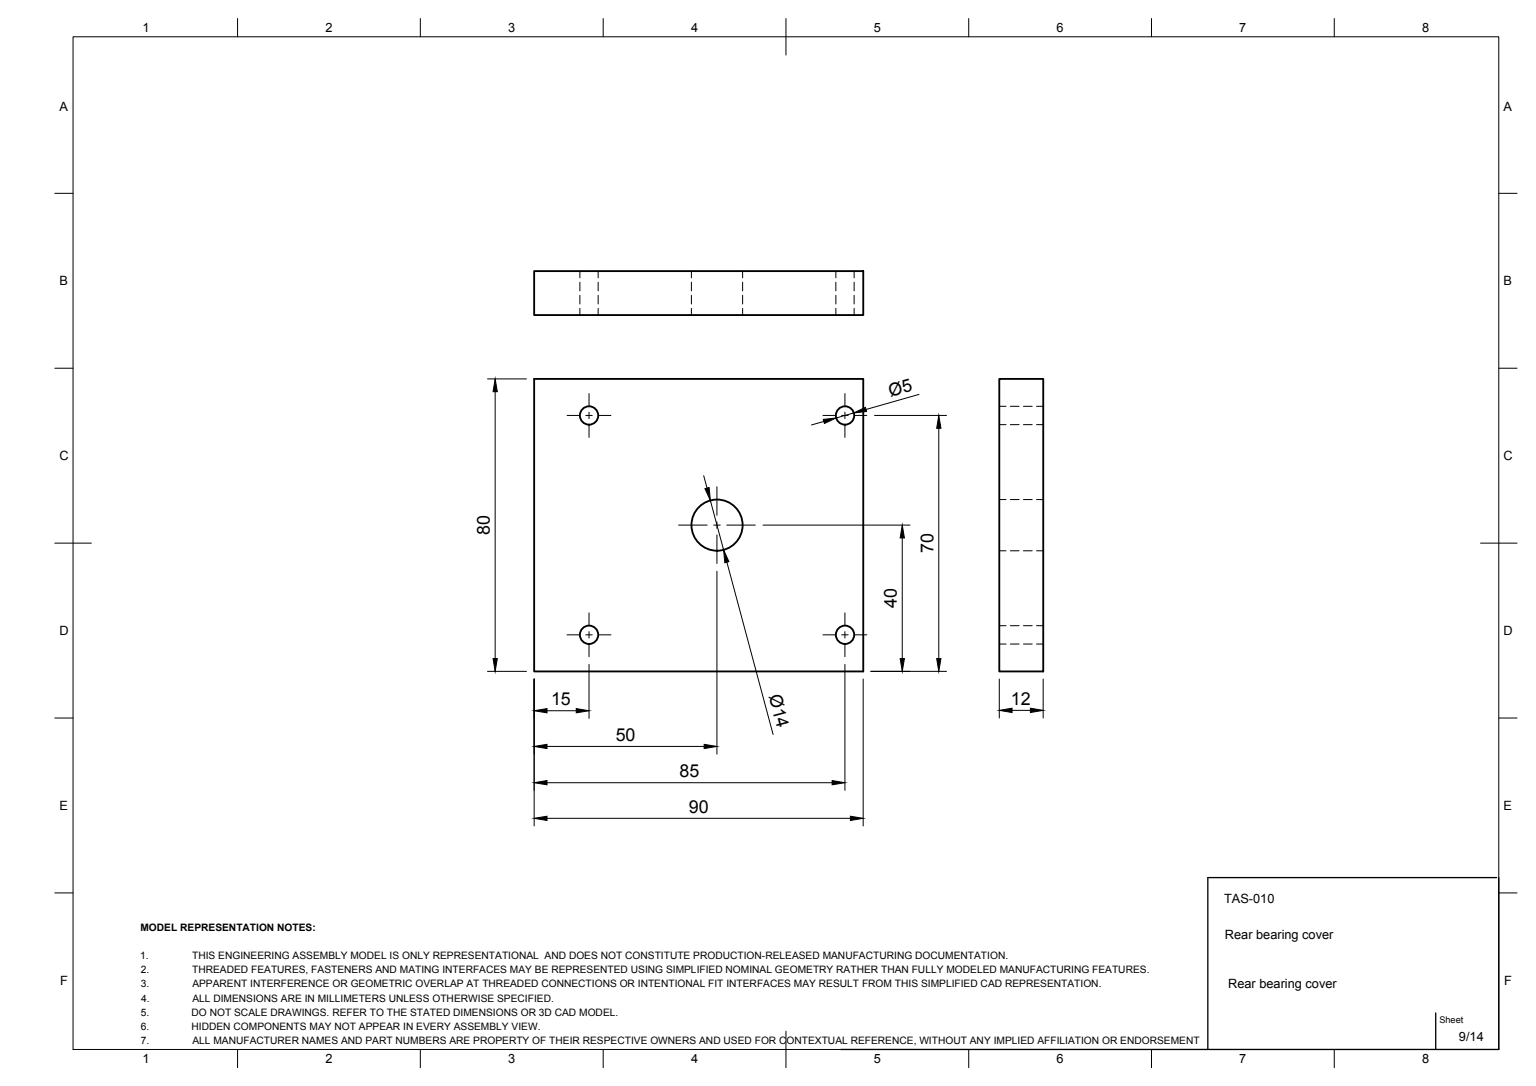
ISO-10303-21;
HEADER;
/* Generated by software containing ST-Developer
 * from STEP Tools, Inc. (www.steptools.com) 
 */

FILE_DESCRIPTION(
/* description */ (
'Independent keyed-quill tailstock, native coupled50mm slider andM16x2
 feed screw, conical dead center, bronze sleeves/thrust washers, cross
-pinned handwheel and bolted guide key. Custom center taper; no standa
rd taper compatibility, machine-bed compatibility or load rating assig
ned.'),
/* implementation_level */ '2;1');

FILE_NAME(
/* name */ 'Rear bearing cover.step',
/* time_stamp */ '2026-11-14T07:17:36-08:00',
/* author */ (''),
/* organization */ (''),
/* preprocessor_version */ 'ST-DEVELOPER v20.2',
/* originating_system */ 'Autodesk Translation Framework v15.17.0.0',
/* authorisation */ '');

FILE_SCHEMA (('AUTOMOTIVE_DESIGN { 1 0 10303 214 3 1 1 }'));
ENDSEC;

DATA;
#10=MECHANICAL_DESIGN_GEOMETRIC_PRESENTATION_REPRESENTATION('',(#159),#289387);
#125=SHAPE_REPRESENTATION_RELATIONSHIP('SRR','None',#289460,#142);
#142=ADVANCED_BREP_SHAPE_REPRESENTATION('',(#176),#289376);
#159=STYLED_ITEM('',(#289552),#176);
#176=MANIFOLD_SOLID_BREP('Body1',#16847);
#228=FACE_BOUND('',#1545,.T.);
#229=FACE_BOUND('',#1546,.T.);
#230=FACE_BOUND('',#1547,.T.);
#231=FACE_BOUND('',#1548,.T.);
#232=FACE_BOUND('',#1549,.T.);
#233=FACE_BOUND('',#1558,.T.);
#234=FACE_BOUND('',#1559,.T.);
#235=FACE_BOUND('',#1560,.T.);
#236=FACE_BOUND('',#1561,.T.);
#237=FACE_BOUND('',#1562,.T.);
#365=PLANE('',#17554);
#366=PLANE('',#17555);
#367=PLANE('',#17556);
#368=PLANE('',#17572);
#369=PLANE('',#17573);
#370=PLANE('',#17574);
#851=FACE_OUTER_BOUND('',#1542,.T.);
#852=FACE_OUTER_BOUND('',#1543,.T.);
#853=FACE_OUTER_BOUND('',#1544,.T.);
#854=FACE_OUTER_BOUND('',#1550,.T.);
#855=FACE_OUTER_BOUND('',#1551,.T.);
#856=FACE_OUTER_BOUND('',#1552,.T.);
#857=FACE_OUTER_BOUND('',#1553,.T.);
#858=FACE_OUTER_BOUND('',#1554,.T.);
#859=FACE_OUTER_BOUND('',#1555,.T.);
#860=FACE_OUTER_BOUND('',#1556,.T.);
#861=FACE_OUTER_BOUND('',#1557,.T.);
#1542=EDGE_LOOP('',(#13733,#13734,#13735,#13736));
#1543=EDGE_LOOP('',(#13737,#13738,#13739,#13740));
#1544=EDGE_LOOP('',(#13741,#13742,#13743,#13744));
#1545=EDGE_LOOP('',(#13745));
#1546=EDGE_LOOP('',(#13746));
#1547=EDGE_LOOP('',(#13747));
#1548=EDGE_LOOP('',(#13748));
#1549=EDGE_LOOP('',(#13749));
#1550=EDGE_LOOP('',(#13750,#13751,#13752,#13753));
#1551=EDGE_LOOP('',(#13754,#13755,#13756,#13757));
#1552=EDGE_LOOP('',(#13758,#13759,#13760,#13761));
#1553=EDGE_LOOP('',(#13762,#13763,#13764,#13765));
#1554=EDGE_LOOP('',(#13766,#13767,#13768,#13769));
#1555=EDGE_LOOP('',(#13770,#13771,#13772,#13773));
#1556=EDGE_LOOP('',(#13774,#13775,#13776,#13777));
#1557=EDGE_LOOP('',(#13778,#13779,#13780,#13781));
#1558=EDGE_LOOP('',(#13782));
#1559=EDGE_LOOP('',(#13783));
#1560=EDGE_LOOP('',(#13784));
#1561=EDGE_LOOP('',(#13785));
#1562=EDGE_LOOP('',(#13786));
#1903=CIRCLE('',#17557,2.5);
#1904=CIRCLE('',#17558,2.5);
#1905=CIRCLE('',#17559,2.5);
#1906=CIRCLE('',#17560,2.5);
#1907=CIRCLE('',#17561,7.);
#1908=CIRCLE('',#17563,2.5);
#1909=CIRCLE('',#17565,2.5);
#1910=CIRCLE('',#17567,2.5);
#1911=CIRCLE('',#17569,2.5);
#1912=CIRCLE('',#17571,7.);
#4355=LINE('',#185232,#4992);
#4356=LINE('',#185234,#4993);
#4357=LINE('',#185236,#4994);
#4358=LINE('',#185237,#4995);
#4359=LINE('',#185240,#4996);
#4360=LINE('',#185242,#4997);
#4361=LINE('',#185243,#4998);
#4362=LINE('',#185246,#4999);
#4363=LINE('',#185247,#5000);
#4364=LINE('',#185261,#5001);
#4365=LINE('',#185265,#5002);
#4366=LINE('',#185269,#5003);
#4367=LINE('',#185273,#5004);
#4368=LINE('',#185277,#5005);
#4369=LINE('',#185280,#5006);
#4370=LINE('',#185281,#5007);
#4371=LINE('',#185283,#5008);
#4992=VECTOR('',#19321,10.);
#4993=VECTOR('',#19322,10.);
#4994=VECTOR('',#19323,10.);
#4995=VECTOR('',#19324,10.);
#4996=VECTOR('',#19327,10.);
#4997=VECTOR('',#19328,10.);
#4998=VECTOR('',#19329,10.);
#4999=VECTOR('',#19332,10.);
#5000=VECTOR('',#19333,10.);
#5001=VECTOR('',#19348,2.5);
#5002=VECTOR('',#19353,2.5);
#5003=VECTOR('',#19358,2.5);
#5004=VECTOR('',#19363,2.5);
#5005=VECTOR('',#19368,7.);
#5006=VECTOR('',#19371,10.);
#5007=VECTOR('',#19372,10.);
#5008=VECTOR('',#19375,10.);
#6600=VERTEX_POINT('',#185230);
#6601=VERTEX_POINT('',#185231);
#6602=VERTEX_POINT('',#185233);
#6603=VERTEX_POINT('',#185235);
#6604=VERTEX_POINT('',#185239);
#6605=VERTEX_POINT('',#185241);
#6606=VERTEX_POINT('',#185245);
#6607=VERTEX_POINT('',#185248);
#6608=VERTEX_POINT('',#185250);
#6609=VERTEX_POINT('',#185252);
#6610=VERTEX_POINT('',#185254);
#6611=VERTEX_POINT('',#185256);
#6612=VERTEX_POINT('',#185259);
#6613=VERTEX_POINT('',#185263);
#6614=VERTEX_POINT('',#185267);
#6615=VERTEX_POINT('',#185271);
#6616=VERTEX_POINT('',#185275);
#6617=VERTEX_POINT('',#185279);
#9178=EDGE_CURVE('',#6600,#6601,#4355,.T.);
#9179=EDGE_CURVE('',#6602,#6600,#4356,.T.);
#9180=EDGE_CURVE('',#6603,#6602,#4357,.T.);
#9181=EDGE_CURVE('',#6601,#6603,#4358,.T.);
#9182=EDGE_CURVE('',#6603,#6604,#4359,.T.);
#9183=EDGE_CURVE('',#6604,#6605,#4360,.T.);
#9184=EDGE_CURVE('',#6601,#6605,#4361,.T.);
#9185=EDGE_CURVE('',#6606,#6602,#4362,.T.);
#9186=EDGE_CURVE('',#6604,#6606,#4363,.T.);
#9187=EDGE_CURVE('',#6607,#6607,#1903,.T.);
#9188=EDGE_CURVE('',#6608,#6608,#1904,.T.);
#9189=EDGE_CURVE('',#6609,#6609,#1905,.T.);
#9190=EDGE_CURVE('',#6610,#6610,#1906,.T.);
#9191=EDGE_CURVE('',#6611,#6611,#1907,.T.);
#9192=EDGE_CURVE('',#6612,#6612,#1908,.T.);
#9193=EDGE_CURVE('',#6612,#6607,#4364,.T.);
#9194=EDGE_CURVE('',#6613,#6613,#1909,.T.);
#9195=EDGE_CURVE('',#6613,#6608,#4365,.T.);
#9196=EDGE_CURVE('',#6614,#6614,#1910,.T.);
#9197=EDGE_CURVE('',#6614,#6609,#4366,.T.);
#9198=EDGE_CURVE('',#6615,#6615,#1911,.T.);
#9199=EDGE_CURVE('',#6615,#6610,#4367,.T.);
#9200=EDGE_CURVE('',#6616,#6616,#1912,.T.);
#9201=EDGE_CURVE('',#6616,#6611,#4368,.T.);
#9202=EDGE_CURVE('',#6606,#6617,#4369,.T.);
#9203=EDGE_CURVE('',#6605,#6617,#4370,.T.);
#9204=EDGE_CURVE('',#6617,#6600,#4371,.T.);
#13733=ORIENTED_EDGE('',*,*,#9178,.F.);
#13734=ORIENTED_EDGE('',*,*,#9179,.F.);
#13735=ORIENTED_EDGE('',*,*,#9180,.F.);
#13736=ORIENTED_EDGE('',*,*,#9181,.F.);
#13737=ORIENTED_EDGE('',*,*,#9181,.T.);
#13738=ORIENTED_EDGE('',*,*,#9182,.T.);
#13739=ORIENTED_EDGE('',*,*,#9183,.T.);
#13740=ORIENTED_EDGE('',*,*,#9184,.F.);
#13741=ORIENTED_EDGE('',*,*,#9180,.T.);
#13742=ORIENTED_EDGE('',*,*,#9185,.F.);
#13743=ORIENTED_EDGE('',*,*,#9186,.F.);
#13744=ORIENTED_EDGE('',*,*,#9182,.F.);
#13745=ORIENTED_EDGE('',*,*,#9187,.T.);
#13746=ORIENTED_EDGE('',*,*,#9188,.T.);
#13747=ORIENTED_EDGE('',*,*,#9189,.T.);
#13748=ORIENTED_EDGE('',*,*,#9190,.T.);
#13749=ORIENTED_EDGE('',*,*,#9191,.T.);
#13750=ORIENTED_EDGE('',*,*,#9192,.F.);
#13751=ORIENTED_EDGE('',*,*,#9193,.T.);
#13752=ORIENTED_EDGE('',*,*,#9187,.F.);
#13753=ORIENTED_EDGE('',*,*,#9193,.F.);
#13754=ORIENTED_EDGE('',*,*,#9194,.F.);
#13755=ORIENTED_EDGE('',*,*,#9195,.T.);
#13756=ORIENTED_EDGE('',*,*,#9188,.F.);
#13757=ORIENTED_EDGE('',*,*,#9195,.F.);
#13758=ORIENTED_EDGE('',*,*,#9196,.F.);
#13759=ORIENTED_EDGE('',*,*,#9197,.T.);
#13760=ORIENTED_EDGE('',*,*,#9189,.F.);
#13761=ORIENTED_EDGE('',*,*,#9197,.F.);
#13762=ORIENTED_EDGE('',*,*,#9198,.F.);
#13763=ORIENTED_EDGE('',*,*,#9199,.T.);
#13764=ORIENTED_EDGE('',*,*,#9190,.F.);
#13765=ORIENTED_EDGE('',*,*,#9199,.F.);
#13766=ORIENTED_EDGE('',*,*,#9200,.F.);
#13767=ORIENTED_EDGE('',*,*,#9201,.T.);
#13768=ORIENTED_EDGE('',*,*,#9191,.F.);
#13769=ORIENTED_EDGE('',*,*,#9201,.F.);
#13770=ORIENTED_EDGE('',*,*,#9186,.T.);
#13771=ORIENTED_EDGE('',*,*,#9202,.T.);
#13772=ORIENTED_EDGE('',*,*,#9203,.F.);
#13773=ORIENTED_EDGE('',*,*,#9183,.F.);
#13774=ORIENTED_EDGE('',*,*,#9179,.T.);
#13775=ORIENTED_EDGE('',*,*,#9204,.F.);
#13776=ORIENTED_EDGE('',*,*,#9202,.F.);
#13777=ORIENTED_EDGE('',*,*,#9185,.T.);
#13778=ORIENTED_EDGE('',*,*,#9178,.T.);
#13779=ORIENTED_EDGE('',*,*,#9184,.T.);
#13780=ORIENTED_EDGE('',*,*,#9203,.T.);
#13781=ORIENTED_EDGE('',*,*,#9204,.T.);
#13782=ORIENTED_EDGE('',*,*,#9200,.T.);
#13783=ORIENTED_EDGE('',*,*,#9198,.T.);
#13784=ORIENTED_EDGE('',*,*,#9196,.T.);
#13785=ORIENTED_EDGE('',*,*,#9194,.T.);
#13786=ORIENTED_EDGE('',*,*,#9192,.T.);
#16040=CYLINDRICAL_SURFACE('',#17562,2.5);
#16041=CYLINDRICAL_SURFACE('',#17564,2.5);
#16042=CYLINDRICAL_SURFACE('',#17566,2.5);
#16043=CYLINDRICAL_SURFACE('',#17568,2.5);
#16044=CYLINDRICAL_SURFACE('',#17570,7.);
#16619=ADVANCED_FACE('',(#851),#365,.F.);
#16620=ADVANCED_FACE('',(#852),#366,.T.);
#16621=ADVANCED_FACE('',(#853,#228,#229,#230,#231,#232),#367,.F.);
#16622=ADVANCED_FACE('',(#854),#16040,.F.);
#16623=ADVANCED_FACE('',(#855),#16041,.F.);
#16624=ADVANCED_FACE('',(#856),#16042,.F.);
#16625=ADVANCED_FACE('',(#857),#16043,.F.);
#16626=ADVANCED_FACE('',(#858),#16044,.F.);
#16627=ADVANCED_FACE('',(#859),#368,.T.);
#16628=ADVANCED_FACE('',(#860),#369,.T.);
#16629=ADVANCED_FACE('',(#861,#233,#234,#235,#236,#237),#370,.T.);
#16847=CLOSED_SHELL('',(#16619,#16620,#16621,#16622,#16623,#16624,#16625,
#16626,#16627,#16628,#16629));
#17553=AXIS2_PLACEMENT_3D('',#185228,#19317,#19318);
#17554=AXIS2_PLACEMENT_3D('',#185229,#19319,#19320);
#17555=AXIS2_PLACEMENT_3D('',#185238,#19325,#19326);
#17556=AXIS2_PLACEMENT_3D('',#185244,#19330,#19331);
#17557=AXIS2_PLACEMENT_3D('',#185249,#19334,#19335);
#17558=AXIS2_PLACEMENT_3D('',#185251,#19336,#19337);
#17559=AXIS2_PLACEMENT_3D('',#185253,#19338,#19339);
#17560=AXIS2_PLACEMENT_3D('',#185255,#19340,#19341);
#17561=AXIS2_PLACEMENT_3D('',#185257,#19342,#19343);
#17562=AXIS2_PLACEMENT_3D('',#185258,#19344,#19345);
#17563=AXIS2_PLACEMENT_3D('',#185260,#19346,#19347);
#17564=AXIS2_PLACEMENT_3D('',#185262,#19349,#19350);
#17565=AXIS2_PLACEMENT_3D('',#185264,#19351,#19352);
#17566=AXIS2_PLACEMENT_3D('',#185266,#19354,#19355);
#17567=AXIS2_PLACEMENT_3D('',#185268,#19356,#19357);
#17568=AXIS2_PLACEMENT_3D('',#185270,#19359,#19360);
#17569=AXIS2_PLACEMENT_3D('',#185272,#19361,#19362);
#17570=AXIS2_PLACEMENT_3D('',#185274,#19364,#19365);
#17571=AXIS2_PLACEMENT_3D('',#185276,#19366,#19367);
#17572=AXIS2_PLACEMENT_3D('',#185278,#19369,#19370);
#17573=AXIS2_PLACEMENT_3D('',#185282,#19373,#19374);
#17574=AXIS2_PLACEMENT_3D('',#185284,#19376,#19377);
#19317=DIRECTION('axis',(0.,0.,1.));
#19318=DIRECTION('refdir',(1.,0.,0.));
#19319=DIRECTION('center_axis',(0.,1.,0.));
#19320=DIRECTION('ref_axis',(1.,0.,0.));
#19321=DIRECTION('',(1.,0.,0.));
#19322=DIRECTION('',(0.,0.,1.));
#19323=DIRECTION('',(-1.,0.,0.));
#19324=DIRECTION('',(0.,0.,-1.));
#19325=DIRECTION('center_axis',(1.,0.,0.));
#19326=DIRECTION('ref_axis',(0.,1.,0.));
#19327=DIRECTION('',(0.,1.,0.));
#19328=DIRECTION('',(0.,0.,1.));
#19329=DIRECTION('',(0.,1.,0.));
#19330=DIRECTION('center_axis',(0.,0.,1.));
#19331=DIRECTION('ref_axis',(1.,0.,0.));
#19332=DIRECTION('',(0.,-1.,0.));
#19333=DIRECTION('',(-1.,0.,0.));
#19334=DIRECTION('center_axis',(0.,0.,1.));
#19335=DIRECTION('ref_axis',(1.,0.,0.));
#19336=DIRECTION('center_axis',(0.,0.,1.));
#19337=DIRECTION('ref_axis',(1.,0.,0.));
#19338=DIRECTION('center_axis',(0.,0.,1.));
#19339=DIRECTION('ref_axis',(1.,0.,0.));
#19340=DIRECTION('center_axis',(0.,0.,1.));
#19341=DIRECTION('ref_axis',(1.,0.,0.));
#19342=DIRECTION('center_axis',(0.,0.,1.));
#19343=DIRECTION('ref_axis',(1.,0.,0.));
#19344=DIRECTION('center_axis',(0.,0.,-1.));
#19345=DIRECTION('ref_axis',(1.,0.,0.));
#19346=DIRECTION('center_axis',(0.,0.,-1.));
#19347=DIRECTION('ref_axis',(1.,0.,0.));
#19348=DIRECTION('',(0.,0.,-1.));
#19349=DIRECTION('center_axis',(0.,0.,-1.));
#19350=DIRECTION('ref_axis',(1.,0.,0.));
#19351=DIRECTION('center_axis',(0.,0.,-1.));
#19352=DIRECTION('ref_axis',(1.,0.,0.));
#19353=DIRECTION('',(0.,0.,-1.));
#19354=DIRECTION('center_axis',(0.,0.,-1.));
#19355=DIRECTION('ref_axis',(1.,0.,0.));
#19356=DIRECTION('center_axis',(0.,0.,-1.));
#19357=DIRECTION('ref_axis',(1.,0.,0.));
#19358=DIRECTION('',(0.,0.,-1.));
#19359=DIRECTION('center_axis',(0.,0.,-1.));
#19360=DIRECTION('ref_axis',(1.,0.,0.));
#19361=DIRECTION('center_axis',(0.,0.,-1.));
#19362=DIRECTION('ref_axis',(1.,0.,0.));
#19363=DIRECTION('',(0.,0.,-1.));
#19364=DIRECTION('center_axis',(0.,0.,-1.));
#19365=DIRECTION('ref_axis',(1.,0.,0.));
#19366=DIRECTION('center_axis',(0.,0.,-1.));
#19367=DIRECTION('ref_axis',(1.,0.,0.));
#19368=DIRECTION('',(0.,0.,-1.));
#19369=DIRECTION('center_axis',(0.,1.,0.));
#19370=DIRECTION('ref_axis',(-1.,0.,0.));
#19371=DIRECTION('',(0.,0.,1.));
#19372=DIRECTION('',(-1.,0.,0.));
#19373=DIRECTION('center_axis',(-1.,0.,0.));
#19374=DIRECTION('ref_axis',(0.,-1.,0.));
#19375=DIRECTION('',(0.,-1.,0.));
#19376=DIRECTION('center_axis',(0.,0.,1.));
#19377=DIRECTION('ref_axis',(1.,0.,0.));
#185228=CARTESIAN_POINT('',(0.,0.,0.));
#185229=CARTESIAN_POINT('Origin',(-40.,-40.,12.));
#185230=CARTESIAN_POINT('',(-40.,-40.,12.));
#185231=CARTESIAN_POINT('',(40.,-40.,12.));
#185232=CARTESIAN_POINT('',(-20.,-40.,12.));
#185233=CARTESIAN_POINT('',(-40.,-40.,0.));
#185234=CARTESIAN_POINT('',(-40.,-40.,6.));
#185235=CARTESIAN_POINT('',(40.,-40.,0.));
#185236=CARTESIAN_POINT('',(-20.,-40.,0.));
#185237=CARTESIAN_POINT('',(40.,-40.,6.));
#185238=CARTESIAN_POINT('Origin',(40.,-50.,0.));
#185239=CARTESIAN_POINT('',(40.,50.,0.));
#185240=CARTESIAN_POINT('',(40.,-50.,0.));
#185241=CARTESIAN_POINT('',(40.,50.,12.));
#185242=CARTESIAN_POINT('',(40.,50.,0.));
#185243=CARTESIAN_POINT('',(40.,-50.,12.));
#185244=CARTESIAN_POINT('Origin',(0.,0.,0.));
#185245=CARTESIAN_POINT('',(-40.,50.,0.));
#185246=CARTESIAN_POINT('',(-40.,50.,0.));
#185247=CARTESIAN_POINT('',(40.,50.,0.));
#185248=CARTESIAN_POINT('',(27.5,-35.,0.));
#185249=CARTESIAN_POINT('Origin',(30.,-35.,0.));
#185250=CARTESIAN_POINT('',(-32.5,-35.,0.));
#185251=CARTESIAN_POINT('Origin',(-30.,-35.,0.));
#185252=CARTESIAN_POINT('',(-32.5,35.,0.));
#185253=CARTESIAN_POINT('Origin',(-30.,35.,0.));
#185254=CARTESIAN_POINT('',(27.5,35.,0.));
#185255=CARTESIAN_POINT('Origin',(30.,35.,0.));
#185256=CARTESIAN_POINT('',(-7.,8.57252759403147E-16,0.));
#185257=CARTESIAN_POINT('Origin',(0.,0.,0.));
#185258=CARTESIAN_POINT('Origin',(30.,-35.,6.));
#185259=CARTESIAN_POINT('',(27.5,-35.,12.));
#185260=CARTESIAN_POINT('Origin',(30.,-35.,12.));
#185261=CARTESIAN_POINT('',(27.5,-35.,6.));
#185262=CARTESIAN_POINT('Origin',(-30.,-35.,6.));
#185263=CARTESIAN_POINT('',(-32.5,-35.,12.));
#185264=CARTESIAN_POINT('Origin',(-30.,-35.,12.));
#185265=CARTESIAN_POINT('',(-32.5,-35.,6.));
#185266=CARTESIAN_POINT('Origin',(-30.,35.,6.));
#185267=CARTESIAN_POINT('',(-32.5,35.,12.));
#185268=CARTESIAN_POINT('Origin',(-30.,35.,12.));
#185269=CARTESIAN_POINT('',(-32.5,35.,6.));
#185270=CARTESIAN_POINT('Origin',(30.,35.,6.));
#185271=CARTESIAN_POINT('',(27.5,35.,12.));
#185272=CARTESIAN_POINT('Origin',(30.,35.,12.));
#185273=CARTESIAN_POINT('',(27.5,35.,6.));
#185274=CARTESIAN_POINT('Origin',(0.,0.,6.));
#185275=CARTESIAN_POINT('',(-7.,8.57252759403147E-16,12.));
#185276=CARTESIAN_POINT('Origin',(0.,0.,12.));
#185277=CARTESIAN_POINT('',(-7.,8.57252759403147E-16,6.));
#185278=CARTESIAN_POINT('Origin',(40.,50.,0.));
#185279=CARTESIAN_POINT('',(-40.,50.,12.));
#185280=CARTESIAN_POINT('',(-40.,50.,0.));
#185281=CARTESIAN_POINT('',(40.,50.,12.));
#185282=CARTESIAN_POINT('Origin',(-40.,50.,0.));
#185283=CARTESIAN_POINT('',(-40.,50.,12.));
#185284=CARTESIAN_POINT('Origin',(0.,0.,12.));
#289357=UNCERTAINTY_MEASURE_WITH_UNIT(LENGTH_MEASURE(0.01),#289388,
'DISTANCE_ACCURACY_VALUE',
'Maximum model space distance between geometric entities at asserted c
onnectivities');
#289368=UNCERTAINTY_MEASURE_WITH_UNIT(LENGTH_MEASURE(0.01),#289388,
'DISTANCE_ACCURACY_VALUE',
'Maximum model space distance between geometric entities at asserted c
onnectivities');
#289376=(
GEOMETRIC_REPRESENTATION_CONTEXT(3)
GLOBAL_UNCERTAINTY_ASSIGNED_CONTEXT((#289357))
GLOBAL_UNIT_ASSIGNED_CONTEXT((#289388,#289390,#289391))
REPRESENTATION_CONTEXT('','3D')
);
#289387=(
GEOMETRIC_REPRESENTATION_CONTEXT(3)
GLOBAL_UNCERTAINTY_ASSIGNED_CONTEXT((#289368))
GLOBAL_UNIT_ASSIGNED_CONTEXT((#289388,#289390,#289391))
REPRESENTATION_CONTEXT('','3D')
);
#289388=(
LENGTH_UNIT()
NAMED_UNIT(*)
SI_UNIT(.MILLI.,.METRE.)
);
#289390=(
NAMED_UNIT(*)
PLANE_ANGLE_UNIT()
SI_UNIT($,.RADIAN.)
);
#289391=(
NAMED_UNIT(*)
SI_UNIT($,.STERADIAN.)
SOLID_ANGLE_UNIT()
);
#289399=SHAPE_DEFINITION_REPRESENTATION(#289417,#289460);
#289417=PRODUCT_DEFINITION_SHAPE('',$,#289479);
#289460=SHAPE_REPRESENTATION('',(#17553),#289376);
#289471=PRODUCT_DEFINITION_CONTEXT('part definition',#289527,'design');
#289479=PRODUCT_DEFINITION('Rear bearing cover','Rear bearing cover',#289497,
#289471);
#289497=PRODUCT_DEFINITION_FORMATION('',$,#289536);
#289527=APPLICATION_CONTEXT(
'Core Data for Automotive Mechanical Design Process');
#289528=PRODUCT_CONTEXT('part definition',#289527,'mechanical');
#289536=PRODUCT('Rear bearing cover','Rear bearing cover',$,(#289528));
#289552=PRESENTATION_STYLE_ASSIGNMENT((#289559));
#289559=SURFACE_STYLE_USAGE(.BOTH.,#289566);
#289566=SURFACE_SIDE_STYLE('',(#289573));
#289573=SURFACE_STYLE_FILL_AREA(#289580);
#289580=FILL_AREA_STYLE('Opaque(81,175,227)',(#289587));
#289587=FILL_AREA_STYLE_COLOUR('Opaque(81,175,227)',#289594);
#289594=COLOUR_RGB('Opaque(81,175,227)',0.317647058823529,0.686274509803922,
0.890196078431372);
ENDSEC;
END-ISO-10303-21;
